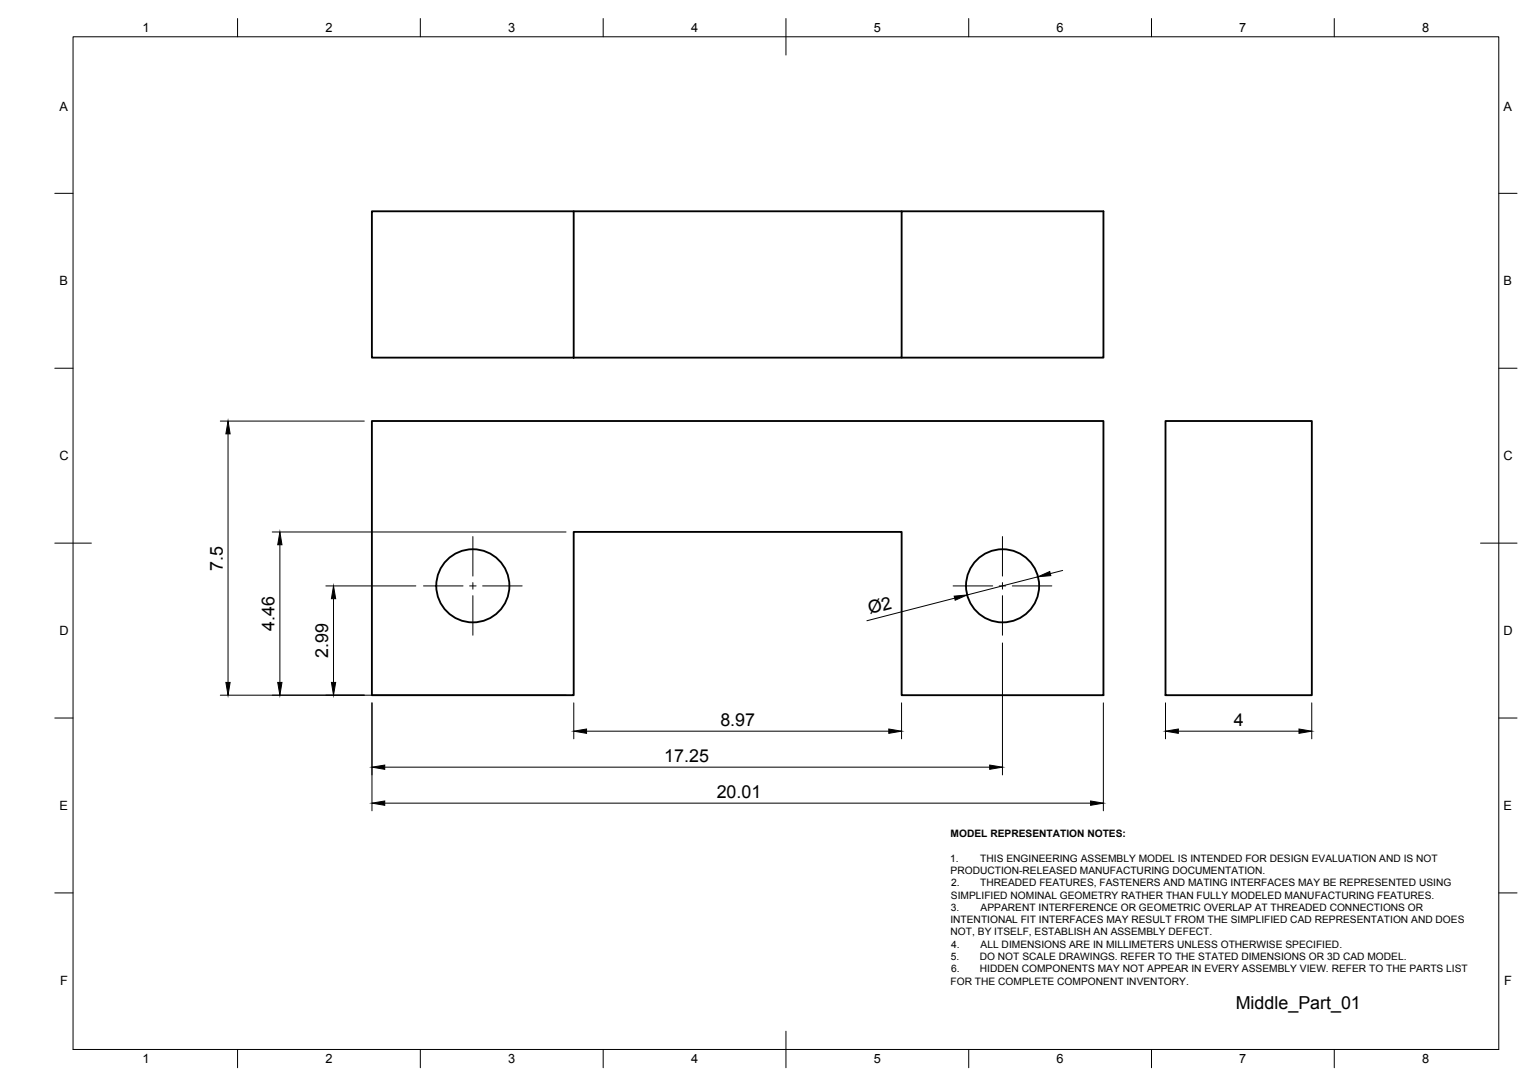
ISO-10303-21;
HEADER;
/* Generated by software containing ST-Developer
 * from STEP Tools, Inc. (www.steptools.com) 
 */

FILE_DESCRIPTION(
/* description */ (''),
/* implementation_level */ '2;1');

FILE_NAME(
/* name */ 'Middle_Part_01.step',
/* time_stamp */ '2026-10-06T13:23:02-07:00',
/* author */ (''),
/* organization */ (''),
/* preprocessor_version */ 'ST-DEVELOPER v20.2',
/* originating_system */ 'Autodesk Translation Framework v15.15.0.0',
/* authorisation */ '');

FILE_SCHEMA (('AUTOMOTIVE_DESIGN { 1 0 10303 214 3 1 1 }'));
ENDSEC;

DATA;
#10=MECHANICAL_DESIGN_GEOMETRIC_PRESENTATION_REPRESENTATION('',(#80),#4994);
#60=SHAPE_REPRESENTATION_RELATIONSHIP('SRR','None',#5041,#70);
#70=ADVANCED_BREP_SHAPE_REPRESENTATION('',(#90),#4993);
#80=STYLED_ITEM('',(#5093),#90);
#90=MANIFOLD_SOLID_BREP('Body1',#2920);
#121=CYLINDRICAL_SURFACE('',#3286,1.);
#122=CYLINDRICAL_SURFACE('',#3289,1.);
#162=FACE_BOUND('',#697,.T.);
#163=FACE_BOUND('',#698,.T.);
#164=FACE_BOUND('',#700,.T.);
#165=FACE_BOUND('',#701,.T.);
#289=PLANE('',#3292);
#290=PLANE('',#3293);
#291=PLANE('',#3294);
#292=PLANE('',#3295);
#293=PLANE('',#3296);
#294=PLANE('',#3297);
#295=PLANE('',#3298);
#296=PLANE('',#3299);
#297=PLANE('',#3300);
#298=PLANE('',#3301);
#469=FACE_OUTER_BOUND('',#686,.T.);
#470=FACE_OUTER_BOUND('',#687,.T.);
#471=FACE_OUTER_BOUND('',#688,.T.);
#472=FACE_OUTER_BOUND('',#689,.T.);
#473=FACE_OUTER_BOUND('',#690,.T.);
#474=FACE_OUTER_BOUND('',#691,.T.);
#475=FACE_OUTER_BOUND('',#692,.T.);
#476=FACE_OUTER_BOUND('',#693,.T.);
#477=FACE_OUTER_BOUND('',#694,.T.);
#478=FACE_OUTER_BOUND('',#695,.T.);
#479=FACE_OUTER_BOUND('',#696,.T.);
#480=FACE_OUTER_BOUND('',#699,.T.);
#686=EDGE_LOOP('',(#2664,#2665,#2666,#2667));
#687=EDGE_LOOP('',(#2668,#2669,#2670,#2671));
#688=EDGE_LOOP('',(#2672,#2673,#2674,#2675));
#689=EDGE_LOOP('',(#2676,#2677,#2678,#2679));
#690=EDGE_LOOP('',(#2680,#2681,#2682,#2683));
#691=EDGE_LOOP('',(#2684,#2685,#2686,#2687));
#692=EDGE_LOOP('',(#2688,#2689,#2690,#2691));
#693=EDGE_LOOP('',(#2692,#2693,#2694,#2695));
#694=EDGE_LOOP('',(#2696,#2697,#2698,#2699));
#695=EDGE_LOOP('',(#2700,#2701,#2702,#2703));
#696=EDGE_LOOP('',(#2704,#2705,#2706,#2707,#2708,#2709,#2710,#2711));
#697=EDGE_LOOP('',(#2712));
#698=EDGE_LOOP('',(#2713));
#699=EDGE_LOOP('',(#2714,#2715,#2716,#2717,#2718,#2719,#2720,#2721));
#700=EDGE_LOOP('',(#2722));
#701=EDGE_LOOP('',(#2723));
#969=LINE('',#4903,#1262);
#970=LINE('',#4909,#1263);
#971=LINE('',#4914,#1264);
#972=LINE('',#4916,#1265);
#973=LINE('',#4918,#1266);
#974=LINE('',#4919,#1267);
#975=LINE('',#4922,#1268);
#976=LINE('',#4924,#1269);
#977=LINE('',#4925,#1270);
#978=LINE('',#4928,#1271);
#979=LINE('',#4930,#1272);
#980=LINE('',#4931,#1273);
#981=LINE('',#4934,#1274);
#982=LINE('',#4936,#1275);
#983=LINE('',#4937,#1276);
#984=LINE('',#4940,#1277);
#985=LINE('',#4942,#1278);
#986=LINE('',#4943,#1279);
#987=LINE('',#4946,#1280);
#988=LINE('',#4948,#1281);
#989=LINE('',#4949,#1282);
#990=LINE('',#4952,#1283);
#991=LINE('',#4954,#1284);
#992=LINE('',#4955,#1285);
#993=LINE('',#4957,#1286);
#994=LINE('',#4958,#1287);
#1262=VECTOR('',#4091,1.);
#1263=VECTOR('',#4098,1.);
#1264=VECTOR('',#4103,10.);
#1265=VECTOR('',#4104,10.);
#1266=VECTOR('',#4105,10.);
#1267=VECTOR('',#4106,10.);
#1268=VECTOR('',#4109,10.);
#1269=VECTOR('',#4110,10.);
#1270=VECTOR('',#4111,10.);
#1271=VECTOR('',#4114,10.);
#1272=VECTOR('',#4115,10.);
#1273=VECTOR('',#4116,10.);
#1274=VECTOR('',#4119,10.);
#1275=VECTOR('',#4120,10.);
#1276=VECTOR('',#4121,10.);
#1277=VECTOR('',#4124,10.);
#1278=VECTOR('',#4125,10.);
#1279=VECTOR('',#4126,10.);
#1280=VECTOR('',#4129,10.);
#1281=VECTOR('',#4130,10.);
#1282=VECTOR('',#4131,10.);
#1283=VECTOR('',#4134,10.);
#1284=VECTOR('',#4135,10.);
#1285=VECTOR('',#4136,10.);
#1286=VECTOR('',#4139,10.);
#1287=VECTOR('',#4140,10.);
#1365=CIRCLE('',#3287,1.);
#1366=CIRCLE('',#3288,1.);
#1367=CIRCLE('',#3290,1.);
#1368=CIRCLE('',#3291,1.);
#1582=VERTEX_POINT('',#4900);
#1583=VERTEX_POINT('',#4902);
#1584=VERTEX_POINT('',#4906);
#1585=VERTEX_POINT('',#4908);
#1586=VERTEX_POINT('',#4912);
#1587=VERTEX_POINT('',#4913);
#1588=VERTEX_POINT('',#4915);
#1589=VERTEX_POINT('',#4917);
#1590=VERTEX_POINT('',#4921);
#1591=VERTEX_POINT('',#4923);
#1592=VERTEX_POINT('',#4927);
#1593=VERTEX_POINT('',#4929);
#1594=VERTEX_POINT('',#4933);
#1595=VERTEX_POINT('',#4935);
#1596=VERTEX_POINT('',#4939);
#1597=VERTEX_POINT('',#4941);
#1598=VERTEX_POINT('',#4945);
#1599=VERTEX_POINT('',#4947);
#1600=VERTEX_POINT('',#4951);
#1601=VERTEX_POINT('',#4953);
#1946=EDGE_CURVE('',#1582,#1582,#1365,.T.);
#1947=EDGE_CURVE('',#1582,#1583,#969,.T.);
#1948=EDGE_CURVE('',#1583,#1583,#1366,.T.);
#1949=EDGE_CURVE('',#1584,#1584,#1367,.T.);
#1950=EDGE_CURVE('',#1584,#1585,#970,.T.);
#1951=EDGE_CURVE('',#1585,#1585,#1368,.T.);
#1952=EDGE_CURVE('',#1586,#1587,#971,.T.);
#1953=EDGE_CURVE('',#1587,#1588,#972,.T.);
#1954=EDGE_CURVE('',#1589,#1588,#973,.T.);
#1955=EDGE_CURVE('',#1586,#1589,#974,.T.);
#1956=EDGE_CURVE('',#1590,#1586,#975,.T.);
#1957=EDGE_CURVE('',#1591,#1589,#976,.T.);
#1958=EDGE_CURVE('',#1590,#1591,#977,.T.);
#1959=EDGE_CURVE('',#1592,#1590,#978,.T.);
#1960=EDGE_CURVE('',#1593,#1591,#979,.T.);
#1961=EDGE_CURVE('',#1592,#1593,#980,.T.);
#1962=EDGE_CURVE('',#1594,#1592,#981,.T.);
#1963=EDGE_CURVE('',#1595,#1593,#982,.T.);
#1964=EDGE_CURVE('',#1594,#1595,#983,.T.);
#1965=EDGE_CURVE('',#1596,#1594,#984,.T.);
#1966=EDGE_CURVE('',#1597,#1595,#985,.T.);
#1967=EDGE_CURVE('',#1596,#1597,#986,.T.);
#1968=EDGE_CURVE('',#1598,#1596,#987,.T.);
#1969=EDGE_CURVE('',#1599,#1597,#988,.T.);
#1970=EDGE_CURVE('',#1598,#1599,#989,.T.);
#1971=EDGE_CURVE('',#1600,#1598,#990,.T.);
#1972=EDGE_CURVE('',#1601,#1599,#991,.T.);
#1973=EDGE_CURVE('',#1600,#1601,#992,.T.);
#1974=EDGE_CURVE('',#1587,#1600,#993,.T.);
#1975=EDGE_CURVE('',#1588,#1601,#994,.T.);
#2664=ORIENTED_EDGE('',*,*,#1946,.F.);
#2665=ORIENTED_EDGE('',*,*,#1947,.T.);
#2666=ORIENTED_EDGE('',*,*,#1948,.F.);
#2667=ORIENTED_EDGE('',*,*,#1947,.F.);
#2668=ORIENTED_EDGE('',*,*,#1949,.F.);
#2669=ORIENTED_EDGE('',*,*,#1950,.T.);
#2670=ORIENTED_EDGE('',*,*,#1951,.F.);
#2671=ORIENTED_EDGE('',*,*,#1950,.F.);
#2672=ORIENTED_EDGE('',*,*,#1952,.T.);
#2673=ORIENTED_EDGE('',*,*,#1953,.T.);
#2674=ORIENTED_EDGE('',*,*,#1954,.F.);
#2675=ORIENTED_EDGE('',*,*,#1955,.F.);
#2676=ORIENTED_EDGE('',*,*,#1956,.T.);
#2677=ORIENTED_EDGE('',*,*,#1955,.T.);
#2678=ORIENTED_EDGE('',*,*,#1957,.F.);
#2679=ORIENTED_EDGE('',*,*,#1958,.F.);
#2680=ORIENTED_EDGE('',*,*,#1959,.T.);
#2681=ORIENTED_EDGE('',*,*,#1958,.T.);
#2682=ORIENTED_EDGE('',*,*,#1960,.F.);
#2683=ORIENTED_EDGE('',*,*,#1961,.F.);
#2684=ORIENTED_EDGE('',*,*,#1962,.T.);
#2685=ORIENTED_EDGE('',*,*,#1961,.T.);
#2686=ORIENTED_EDGE('',*,*,#1963,.F.);
#2687=ORIENTED_EDGE('',*,*,#1964,.F.);
#2688=ORIENTED_EDGE('',*,*,#1965,.T.);
#2689=ORIENTED_EDGE('',*,*,#1964,.T.);
#2690=ORIENTED_EDGE('',*,*,#1966,.F.);
#2691=ORIENTED_EDGE('',*,*,#1967,.F.);
#2692=ORIENTED_EDGE('',*,*,#1968,.T.);
#2693=ORIENTED_EDGE('',*,*,#1967,.T.);
#2694=ORIENTED_EDGE('',*,*,#1969,.F.);
#2695=ORIENTED_EDGE('',*,*,#1970,.F.);
#2696=ORIENTED_EDGE('',*,*,#1971,.T.);
#2697=ORIENTED_EDGE('',*,*,#1970,.T.);
#2698=ORIENTED_EDGE('',*,*,#1972,.F.);
#2699=ORIENTED_EDGE('',*,*,#1973,.F.);
#2700=ORIENTED_EDGE('',*,*,#1974,.T.);
#2701=ORIENTED_EDGE('',*,*,#1973,.T.);
#2702=ORIENTED_EDGE('',*,*,#1975,.F.);
#2703=ORIENTED_EDGE('',*,*,#1953,.F.);
#2704=ORIENTED_EDGE('',*,*,#1975,.T.);
#2705=ORIENTED_EDGE('',*,*,#1972,.T.);
#2706=ORIENTED_EDGE('',*,*,#1969,.T.);
#2707=ORIENTED_EDGE('',*,*,#1966,.T.);
#2708=ORIENTED_EDGE('',*,*,#1963,.T.);
#2709=ORIENTED_EDGE('',*,*,#1960,.T.);
#2710=ORIENTED_EDGE('',*,*,#1957,.T.);
#2711=ORIENTED_EDGE('',*,*,#1954,.T.);
#2712=ORIENTED_EDGE('',*,*,#1946,.T.);
#2713=ORIENTED_EDGE('',*,*,#1949,.T.);
#2714=ORIENTED_EDGE('',*,*,#1974,.F.);
#2715=ORIENTED_EDGE('',*,*,#1952,.F.);
#2716=ORIENTED_EDGE('',*,*,#1956,.F.);
#2717=ORIENTED_EDGE('',*,*,#1959,.F.);
#2718=ORIENTED_EDGE('',*,*,#1962,.F.);
#2719=ORIENTED_EDGE('',*,*,#1965,.F.);
#2720=ORIENTED_EDGE('',*,*,#1968,.F.);
#2721=ORIENTED_EDGE('',*,*,#1971,.F.);
#2722=ORIENTED_EDGE('',*,*,#1948,.T.);
#2723=ORIENTED_EDGE('',*,*,#1951,.T.);
#2899=ADVANCED_FACE('',(#469),#121,.F.);
#2900=ADVANCED_FACE('',(#470),#122,.F.);
#2901=ADVANCED_FACE('',(#471),#289,.T.);
#2902=ADVANCED_FACE('',(#472),#290,.T.);
#2903=ADVANCED_FACE('',(#473),#291,.T.);
#2904=ADVANCED_FACE('',(#474),#292,.T.);
#2905=ADVANCED_FACE('',(#475),#293,.T.);
#2906=ADVANCED_FACE('',(#476),#294,.T.);
#2907=ADVANCED_FACE('',(#477),#295,.T.);
#2908=ADVANCED_FACE('',(#478),#296,.T.);
#2909=ADVANCED_FACE('',(#479,#162,#163),#297,.T.);
#2910=ADVANCED_FACE('',(#480,#164,#165),#298,.F.);
#2920=CLOSED_SHELL('',(#2899,#2900,#2901,#2902,#2903,#2904,#2905,#2906,
#2907,#2908,#2909,#2910));
#3285=AXIS2_PLACEMENT_3D('',#4898,#4085,#4086);
#3286=AXIS2_PLACEMENT_3D('',#4899,#4087,#4088);
#3287=AXIS2_PLACEMENT_3D('',#4901,#4089,#4090);
#3288=AXIS2_PLACEMENT_3D('',#4904,#4092,#4093);
#3289=AXIS2_PLACEMENT_3D('',#4905,#4094,#4095);
#3290=AXIS2_PLACEMENT_3D('',#4907,#4096,#4097);
#3291=AXIS2_PLACEMENT_3D('',#4910,#4099,#4100);
#3292=AXIS2_PLACEMENT_3D('',#4911,#4101,#4102);
#3293=AXIS2_PLACEMENT_3D('',#4920,#4107,#4108);
#3294=AXIS2_PLACEMENT_3D('',#4926,#4112,#4113);
#3295=AXIS2_PLACEMENT_3D('',#4932,#4117,#4118);
#3296=AXIS2_PLACEMENT_3D('',#4938,#4122,#4123);
#3297=AXIS2_PLACEMENT_3D('',#4944,#4127,#4128);
#3298=AXIS2_PLACEMENT_3D('',#4950,#4132,#4133);
#3299=AXIS2_PLACEMENT_3D('',#4956,#4137,#4138);
#3300=AXIS2_PLACEMENT_3D('',#4959,#4141,#4142);
#3301=AXIS2_PLACEMENT_3D('',#4960,#4143,#4144);
#4085=DIRECTION('axis',(0.,0.,1.));
#4086=DIRECTION('refdir',(1.,0.,0.));
#4087=DIRECTION('center_axis',(-1.,0.,0.));
#4088=DIRECTION('ref_axis',(0.,1.,0.));
#4089=DIRECTION('center_axis',(-1.,0.,0.));
#4090=DIRECTION('ref_axis',(0.,1.,0.));
#4091=DIRECTION('',(-1.,0.,0.));
#4092=DIRECTION('center_axis',(1.,0.,0.));
#4093=DIRECTION('ref_axis',(0.,1.,0.));
#4094=DIRECTION('center_axis',(-1.,0.,0.));
#4095=DIRECTION('ref_axis',(0.,1.,0.));
#4096=DIRECTION('center_axis',(-1.,0.,0.));
#4097=DIRECTION('ref_axis',(0.,1.,0.));
#4098=DIRECTION('',(-1.,0.,0.));
#4099=DIRECTION('center_axis',(1.,0.,0.));
#4100=DIRECTION('ref_axis',(0.,1.,0.));
#4101=DIRECTION('center_axis',(0.,0.,1.));
#4102=DIRECTION('ref_axis',(0.,-1.,0.));
#4103=DIRECTION('',(0.,-1.,0.));
#4104=DIRECTION('',(1.,0.,0.));
#4105=DIRECTION('',(0.,-1.,0.));
#4106=DIRECTION('',(1.,0.,0.));
#4107=DIRECTION('center_axis',(0.,1.,0.));
#4108=DIRECTION('ref_axis',(0.,0.,1.));
#4109=DIRECTION('',(0.,0.,1.));
#4110=DIRECTION('',(0.,0.,1.));
#4111=DIRECTION('',(1.,0.,0.));
#4112=DIRECTION('center_axis',(0.,0.,-1.));
#4113=DIRECTION('ref_axis',(0.,1.,0.));
#4114=DIRECTION('',(0.,1.,0.));
#4115=DIRECTION('',(0.,1.,0.));
#4116=DIRECTION('',(1.,0.,0.));
#4117=DIRECTION('center_axis',(0.,-1.,0.));
#4118=DIRECTION('ref_axis',(0.,0.,-1.));
#4119=DIRECTION('',(0.,0.,-1.));
#4120=DIRECTION('',(0.,0.,-1.));
#4121=DIRECTION('',(1.,0.,0.));
#4122=DIRECTION('center_axis',(0.,0.,-1.));
#4123=DIRECTION('ref_axis',(0.,1.,0.));
#4124=DIRECTION('',(0.,1.,0.));
#4125=DIRECTION('',(0.,1.,0.));
#4126=DIRECTION('',(1.,0.,0.));
#4127=DIRECTION('center_axis',(0.,1.,-1.24327477962315E-16));
#4128=DIRECTION('ref_axis',(0.,1.24327477962315E-16,1.));
#4129=DIRECTION('',(0.,1.24327477962315E-16,1.));
#4130=DIRECTION('',(0.,1.24327477962315E-16,1.));
#4131=DIRECTION('',(1.,0.,0.));
#4132=DIRECTION('center_axis',(0.,0.,-1.));
#4133=DIRECTION('ref_axis',(0.,1.,0.));
#4134=DIRECTION('',(0.,1.,0.));
#4135=DIRECTION('',(0.,1.,0.));
#4136=DIRECTION('',(1.,0.,0.));
#4137=DIRECTION('center_axis',(0.,-1.,0.));
#4138=DIRECTION('ref_axis',(0.,0.,-1.));
#4139=DIRECTION('',(0.,0.,-1.));
#4140=DIRECTION('',(0.,0.,-1.));
#4141=DIRECTION('center_axis',(1.,0.,0.));
#4142=DIRECTION('ref_axis',(0.,0.,-1.));
#4143=DIRECTION('center_axis',(1.,0.,0.));
#4144=DIRECTION('ref_axis',(0.,1.,0.));
#4898=CARTESIAN_POINT('',(0.,0.,0.));
#4899=CARTESIAN_POINT('Origin',(14.5,7.24395366693103,1.75498192028357));
#4900=CARTESIAN_POINT('',(13.5,6.24395366693103,1.75498192028357));
#4901=CARTESIAN_POINT('Origin',(13.5,7.24395366693103,1.75498192028357));
#4902=CARTESIAN_POINT('',(9.5,6.24395366693103,1.75498192028357));
#4903=CARTESIAN_POINT('',(14.5,6.24395366693103,1.75498192028357));
#4904=CARTESIAN_POINT('Origin',(9.5,7.24395366693103,1.75498192028357));
#4905=CARTESIAN_POINT('Origin',(14.5,-7.24395366693103,1.75498192028357));
#4906=CARTESIAN_POINT('',(13.5,-8.24395366693103,1.75498192028357));
#4907=CARTESIAN_POINT('Origin',(13.5,-7.24395366693103,1.75498192028357));
#4908=CARTESIAN_POINT('',(9.5,-8.24395366693103,1.75498192028357));
#4909=CARTESIAN_POINT('',(14.5,-8.24395366693103,1.75498192028357));
#4910=CARTESIAN_POINT('Origin',(9.5,-7.24395366693103,1.75498192028357));
#4911=CARTESIAN_POINT('Origin',(9.5,10.0039433906299,6.26348125396711));
#4912=CARTESIAN_POINT('',(9.5,10.0039433906299,6.26348125396711));
#4913=CARTESIAN_POINT('',(9.5,-10.0039433906299,6.26348125396711));
#4914=CARTESIAN_POINT('',(9.5,10.0039433906299,6.26348125396711));
#4915=CARTESIAN_POINT('',(13.5,-10.0039433906299,6.26348125396711));
#4916=CARTESIAN_POINT('',(9.5,-10.0039433906299,6.26348125396711));
#4917=CARTESIAN_POINT('',(13.5,10.0039433906299,6.26348125396711));
#4918=CARTESIAN_POINT('',(13.5,10.0039433906299,6.26348125396711));
#4919=CARTESIAN_POINT('',(9.5,10.0039433906299,6.26348125396711));
#4920=CARTESIAN_POINT('Origin',(9.5,10.0039433906299,-1.2346845122375));
#4921=CARTESIAN_POINT('',(9.5,10.0039433906299,-1.2346845122375));
#4922=CARTESIAN_POINT('',(9.5,10.0039433906299,-1.2346845122375));
#4923=CARTESIAN_POINT('',(13.5,10.0039433906299,-1.2346845122375));
#4924=CARTESIAN_POINT('',(13.5,10.0039433906299,-1.2346845122375));
#4925=CARTESIAN_POINT('',(9.5,10.0039433906299,-1.2346845122375));
#4926=CARTESIAN_POINT('Origin',(9.5,4.48396394323217,-1.2346845122375));
#4927=CARTESIAN_POINT('',(9.5,4.48396394323217,-1.2346845122375));
#4928=CARTESIAN_POINT('',(9.5,-10.0039433906299,-1.2346845122375));
#4929=CARTESIAN_POINT('',(13.5,4.48396394323217,-1.2346845122375));
#4930=CARTESIAN_POINT('',(13.5,-10.0039433906299,-1.2346845122375));
#4931=CARTESIAN_POINT('',(9.5,4.48396394323217,-1.2346845122375));
#4932=CARTESIAN_POINT('Origin',(9.5,4.48396394323217,3.23022961141938));
#4933=CARTESIAN_POINT('',(9.5,4.48396394323217,3.23022961141938));
#4934=CARTESIAN_POINT('',(9.5,4.48396394323217,3.23022961141938));
#4935=CARTESIAN_POINT('',(13.5,4.48396394323217,3.23022961141938));
#4936=CARTESIAN_POINT('',(13.5,4.48396394323217,3.23022961141938));
#4937=CARTESIAN_POINT('',(9.5,4.48396394323217,3.23022961141938));
#4938=CARTESIAN_POINT('Origin',(9.5,-4.48396394323217,3.23022961141938));
#4939=CARTESIAN_POINT('',(9.5,-4.48396394323217,3.23022961141938));
#4940=CARTESIAN_POINT('',(9.5,-4.48396394323217,3.23022961141938));
#4941=CARTESIAN_POINT('',(13.5,-4.48396394323217,3.23022961141938));
#4942=CARTESIAN_POINT('',(13.5,-4.48396394323217,3.23022961141938));
#4943=CARTESIAN_POINT('',(9.5,-4.48396394323217,3.23022961141938));
#4944=CARTESIAN_POINT('Origin',(9.5,-4.48396394323217,-1.2346845122375));
#4945=CARTESIAN_POINT('',(9.5,-4.48396394323217,-1.2346845122375));
#4946=CARTESIAN_POINT('',(9.5,-4.48396394323217,-1.2346845122375));
#4947=CARTESIAN_POINT('',(13.5,-4.48396394323217,-1.2346845122375));
#4948=CARTESIAN_POINT('',(13.5,-4.48396394323217,-1.2346845122375));
#4949=CARTESIAN_POINT('',(9.5,-4.48396394323217,-1.2346845122375));
#4950=CARTESIAN_POINT('Origin',(9.5,-10.0039433906299,-1.2346845122375));
#4951=CARTESIAN_POINT('',(9.5,-10.0039433906299,-1.2346845122375));
#4952=CARTESIAN_POINT('',(9.5,-10.0039433906299,-1.2346845122375));
#4953=CARTESIAN_POINT('',(13.5,-10.0039433906299,-1.2346845122375));
#4954=CARTESIAN_POINT('',(13.5,-10.0039433906299,-1.2346845122375));
#4955=CARTESIAN_POINT('',(9.5,-10.0039433906299,-1.2346845122375));
#4956=CARTESIAN_POINT('Origin',(9.5,-10.0039433906299,6.26348125396711));
#4957=CARTESIAN_POINT('',(9.5,-10.0039433906299,6.26348125396711));
#4958=CARTESIAN_POINT('',(13.5,-10.0039433906299,6.26348125396711));
#4959=CARTESIAN_POINT('Origin',(13.5,0.,2.51439837086481));
#4960=CARTESIAN_POINT('Origin',(9.5,0.,2.51439837086481));
#4981=UNCERTAINTY_MEASURE_WITH_UNIT(LENGTH_MEASURE(0.01),#4995,
'DISTANCE_ACCURACY_VALUE',
'Maximum model space distance between geometric entities at asserted c
onnectivities');
#4982=UNCERTAINTY_MEASURE_WITH_UNIT(LENGTH_MEASURE(0.01),#4995,
'DISTANCE_ACCURACY_VALUE',
'Maximum model space distance between geometric entities at asserted c
onnectivities');
#4993=(
GEOMETRIC_REPRESENTATION_CONTEXT(3)
GLOBAL_UNCERTAINTY_ASSIGNED_CONTEXT((#4981))
GLOBAL_UNIT_ASSIGNED_CONTEXT((#4995,#4997,#4998))
REPRESENTATION_CONTEXT('','3D')
);
#4994=(
GEOMETRIC_REPRESENTATION_CONTEXT(3)
GLOBAL_UNCERTAINTY_ASSIGNED_CONTEXT((#4982))
GLOBAL_UNIT_ASSIGNED_CONTEXT((#4995,#4997,#4998))
REPRESENTATION_CONTEXT('','3D')
);
#4995=(
LENGTH_UNIT()
NAMED_UNIT(*)
SI_UNIT(.MILLI.,.METRE.)
);
#4997=(
NAMED_UNIT(*)
PLANE_ANGLE_UNIT()
SI_UNIT($,.RADIAN.)
);
#4998=(
NAMED_UNIT(*)
SI_UNIT($,.STERADIAN.)
SOLID_ANGLE_UNIT()
);
#5009=SHAPE_DEFINITION_REPRESENTATION(#5020,#5041);
#5020=PRODUCT_DEFINITION_SHAPE('',$,#5053);
#5041=SHAPE_REPRESENTATION('',(#3285),#4993);
#5042=PRODUCT_DEFINITION_CONTEXT('part definition',#5077,'design');
#5053=PRODUCT_DEFINITION('Middle_Part_01','Middle_Part_01',#5064,#5042);
#5064=PRODUCT_DEFINITION_FORMATION('',$,#5089);
#5077=APPLICATION_CONTEXT(
'Core Data for Automotive Mechanical Design Process');
#5078=PRODUCT_CONTEXT('part definition',#5077,'mechanical');
#5089=PRODUCT('Middle_Part_01','Middle_Part_01',$,(#5078));
#5093=PRESENTATION_STYLE_ASSIGNMENT((#5098));
#5098=SURFACE_STYLE_USAGE(.BOTH.,#5103);
#5103=SURFACE_SIDE_STYLE('',(#5108));
#5108=SURFACE_STYLE_FILL_AREA(#5113);
#5113=FILL_AREA_STYLE('Opaque(70,70,209)',(#5118));
#5118=FILL_AREA_STYLE_COLOUR('Opaque(70,70,209)',#5123);
#5123=COLOUR_RGB('Opaque(70,70,209)', 0.09019608, 0.27058824, 0.51372549);
ENDSEC;
END-ISO-10303-21;
